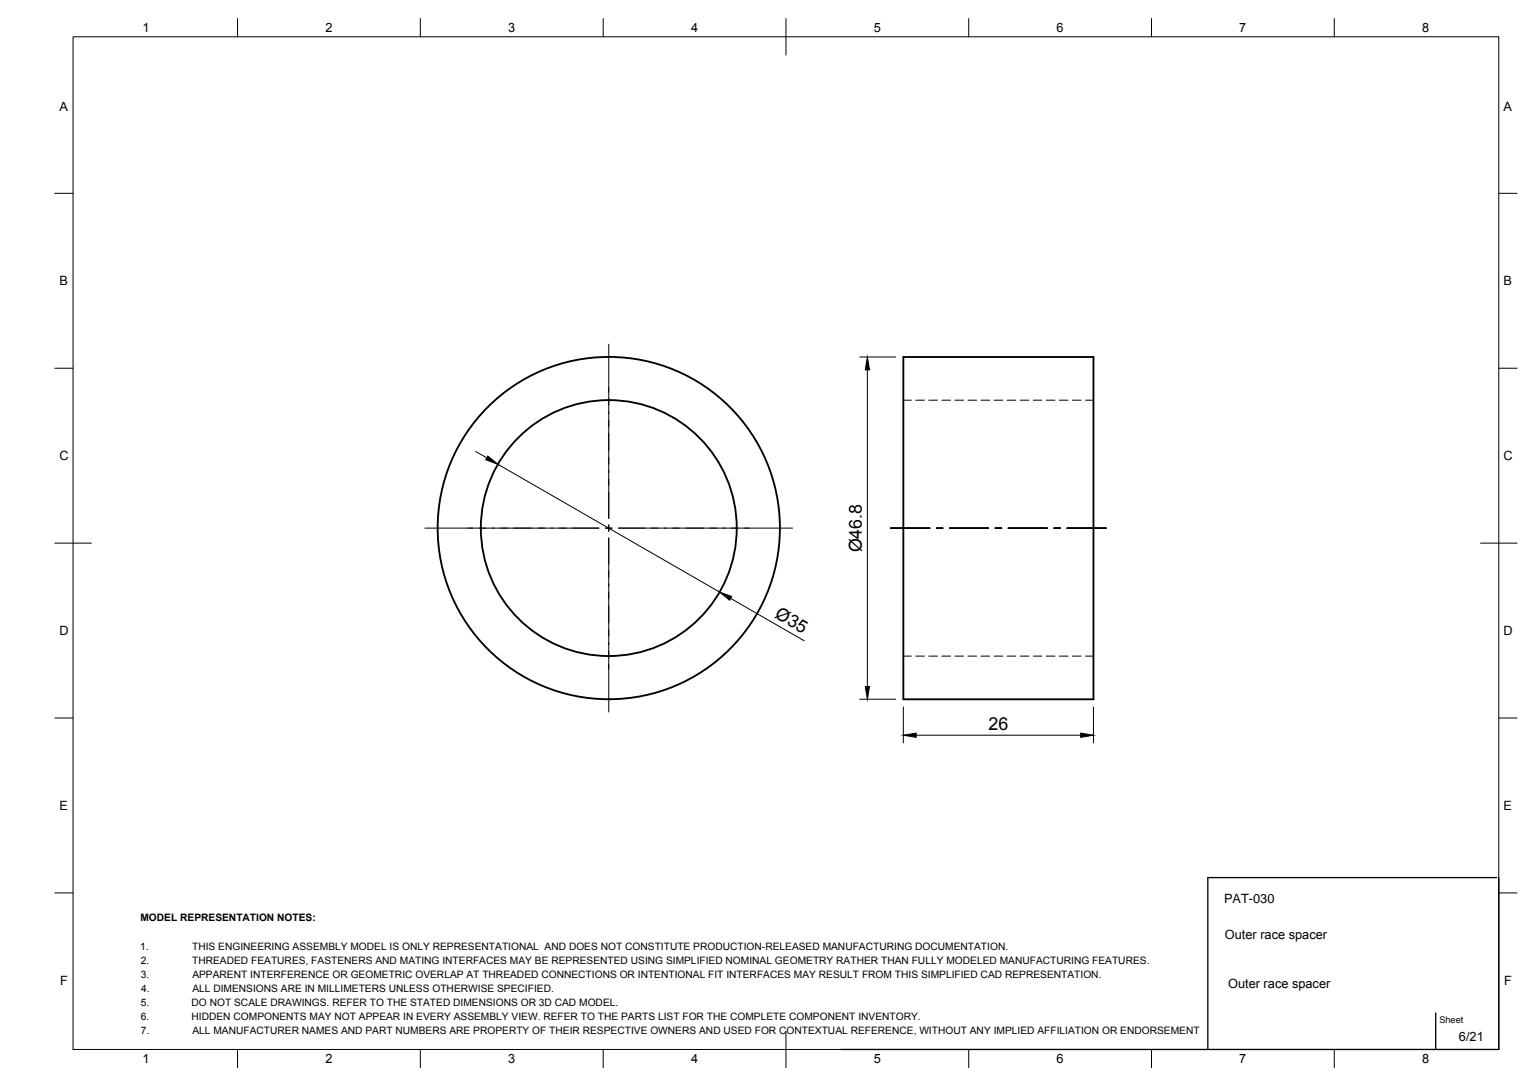
ISO-10303-21;
HEADER;
/* Generated by software containing ST-Developer
 * from STEP Tools, Inc. (www.steptools.com) 
 */

FILE_DESCRIPTION(
/* description */ ('Double-bearing flanged cartridge'),
/* implementation_level */ '2;1');

FILE_NAME(
/* name */ 'Outer race spacer.step',
/* time_stamp */ '2026-10-28T03:26:40-07:00',
/* author */ (''),
/* organization */ (''),
/* preprocessor_version */ 'ST-DEVELOPER v20.2',
/* originating_system */ 'Autodesk Translation Framework v15.17.0.0',
/* authorisation */ '');

FILE_SCHEMA (('AUTOMOTIVE_DESIGN { 1 0 10303 214 3 1 1 }'));
ENDSEC;

DATA;
#10=MECHANICAL_DESIGN_GEOMETRIC_PRESENTATION_REPRESENTATION('',(#204),#5535);
#168=SHAPE_REPRESENTATION_RELATIONSHIP('SRR','None',#5610,#182);
#182=ADVANCED_BREP_SHAPE_REPRESENTATION('',(#226),#5526);
#204=STYLED_ITEM('',(#5764),#226);
#226=MANIFOLD_SOLID_BREP('Body1',#2338);
#262=FACE_BOUND('',#621,.T.);
#263=FACE_BOUND('',#623,.T.);
#329=PLANE('',#2706);
#330=PLANE('',#2707);
#440=FACE_OUTER_BOUND('',#618,.T.);
#441=FACE_OUTER_BOUND('',#619,.T.);
#442=FACE_OUTER_BOUND('',#620,.T.);
#443=FACE_OUTER_BOUND('',#622,.T.);
#618=EDGE_LOOP('',(#1858,#1859,#1860,#1861));
#619=EDGE_LOOP('',(#1862,#1863,#1864,#1865));
#620=EDGE_LOOP('',(#1866));
#621=EDGE_LOOP('',(#1867));
#622=EDGE_LOOP('',(#1868));
#623=EDGE_LOOP('',(#1869));
#758=LINE('',#4385,#844);
#759=LINE('',#4391,#845);
#844=VECTOR('',#3299,1.75);
#845=VECTOR('',#3306,2.34);
#1002=CIRCLE('',#2701,1.75);
#1003=CIRCLE('',#2702,1.75);
#1004=CIRCLE('',#2704,2.34);
#1005=CIRCLE('',#2705,2.34);
#1184=VERTEX_POINT('',#4382);
#1185=VERTEX_POINT('',#4384);
#1186=VERTEX_POINT('',#4388);
#1187=VERTEX_POINT('',#4390);
#1422=EDGE_CURVE('',#1184,#1184,#1002,.T.);
#1423=EDGE_CURVE('',#1184,#1185,#758,.T.);
#1424=EDGE_CURVE('',#1185,#1185,#1003,.T.);
#1425=EDGE_CURVE('',#1186,#1186,#1004,.T.);
#1426=EDGE_CURVE('',#1186,#1187,#759,.T.);
#1427=EDGE_CURVE('',#1187,#1187,#1005,.T.);
#1858=ORIENTED_EDGE('',*,*,#1422,.F.);
#1859=ORIENTED_EDGE('',*,*,#1423,.T.);
#1860=ORIENTED_EDGE('',*,*,#1424,.T.);
#1861=ORIENTED_EDGE('',*,*,#1423,.F.);
#1862=ORIENTED_EDGE('',*,*,#1425,.F.);
#1863=ORIENTED_EDGE('',*,*,#1426,.T.);
#1864=ORIENTED_EDGE('',*,*,#1427,.T.);
#1865=ORIENTED_EDGE('',*,*,#1426,.F.);
#1866=ORIENTED_EDGE('',*,*,#1425,.T.);
#1867=ORIENTED_EDGE('',*,*,#1422,.T.);
#1868=ORIENTED_EDGE('',*,*,#1427,.F.);
#1869=ORIENTED_EDGE('',*,*,#1424,.F.);
#2142=CYLINDRICAL_SURFACE('',#2700,1.75);
#2143=CYLINDRICAL_SURFACE('',#2703,2.34);
#2254=ADVANCED_FACE('',(#440),#2142,.F.);
#2255=ADVANCED_FACE('',(#441),#2143,.T.);
#2256=ADVANCED_FACE('',(#442,#262),#329,.T.);
#2257=ADVANCED_FACE('',(#443,#263),#330,.F.);
#2338=CLOSED_SHELL('',(#2254,#2255,#2256,#2257));
#2699=AXIS2_PLACEMENT_3D('',#4380,#3293,#3294);
#2700=AXIS2_PLACEMENT_3D('',#4381,#3295,#3296);
#2701=AXIS2_PLACEMENT_3D('',#4383,#3297,#3298);
#2702=AXIS2_PLACEMENT_3D('',#4386,#3300,#3301);
#2703=AXIS2_PLACEMENT_3D('',#4387,#3302,#3303);
#2704=AXIS2_PLACEMENT_3D('',#4389,#3304,#3305);
#2705=AXIS2_PLACEMENT_3D('',#4392,#3307,#3308);
#2706=AXIS2_PLACEMENT_3D('',#4393,#3309,#3310);
#2707=AXIS2_PLACEMENT_3D('',#4394,#3311,#3312);
#3293=DIRECTION('axis',(0.,0.,1.));
#3294=DIRECTION('refdir',(1.,0.,0.));
#3295=DIRECTION('center_axis',(0.,1.,0.));
#3296=DIRECTION('ref_axis',(1.,0.,0.));
#3297=DIRECTION('center_axis',(0.,-1.,0.));
#3298=DIRECTION('ref_axis',(1.,0.,0.));
#3299=DIRECTION('',(0.,-1.,0.));
#3300=DIRECTION('center_axis',(0.,-1.,0.));
#3301=DIRECTION('ref_axis',(1.,0.,0.));
#3302=DIRECTION('center_axis',(0.,1.,0.));
#3303=DIRECTION('ref_axis',(1.,0.,0.));
#3304=DIRECTION('center_axis',(0.,1.,0.));
#3305=DIRECTION('ref_axis',(1.,0.,0.));
#3306=DIRECTION('',(0.,-1.,0.));
#3307=DIRECTION('center_axis',(0.,1.,0.));
#3308=DIRECTION('ref_axis',(1.,0.,0.));
#3309=DIRECTION('center_axis',(0.,1.,0.));
#3310=DIRECTION('ref_axis',(1.,0.,0.));
#3311=DIRECTION('center_axis',(0.,1.,0.));
#3312=DIRECTION('ref_axis',(1.,0.,0.));
#4380=CARTESIAN_POINT('',(0.,0.,0.));
#4381=CARTESIAN_POINT('Origin',(0.,1.7,4.5));
#4382=CARTESIAN_POINT('',(-1.75,4.3,4.5));
#4383=CARTESIAN_POINT('Origin',(0.,4.3,4.5));
#4384=CARTESIAN_POINT('',(-1.75,1.7,4.5));
#4385=CARTESIAN_POINT('',(-1.75,1.7,4.5));
#4386=CARTESIAN_POINT('Origin',(0.,1.7,4.5));
#4387=CARTESIAN_POINT('Origin',(0.,1.7,4.5));
#4388=CARTESIAN_POINT('',(-2.34,4.3,4.5));
#4389=CARTESIAN_POINT('Origin',(0.,4.3,4.5));
#4390=CARTESIAN_POINT('',(-2.34,1.7,4.5));
#4391=CARTESIAN_POINT('',(-2.34,1.7,4.5));
#4392=CARTESIAN_POINT('Origin',(0.,1.7,4.5));
#4393=CARTESIAN_POINT('Origin',(0.,4.3,4.5));
#4394=CARTESIAN_POINT('Origin',(0.,1.7,4.5));
#5507=UNCERTAINTY_MEASURE_WITH_UNIT(LENGTH_MEASURE(0.001),#5536,
'DISTANCE_ACCURACY_VALUE',
'Maximum model space distance between geometric entities at asserted c
onnectivities');
#5516=UNCERTAINTY_MEASURE_WITH_UNIT(LENGTH_MEASURE(0.001),#5536,
'DISTANCE_ACCURACY_VALUE',
'Maximum model space distance between geometric entities at asserted c
onnectivities');
#5526=(
GEOMETRIC_REPRESENTATION_CONTEXT(3)
GLOBAL_UNCERTAINTY_ASSIGNED_CONTEXT((#5507))
GLOBAL_UNIT_ASSIGNED_CONTEXT((#5536,#5538,#5539))
REPRESENTATION_CONTEXT('','3D')
);
#5535=(
GEOMETRIC_REPRESENTATION_CONTEXT(3)
GLOBAL_UNCERTAINTY_ASSIGNED_CONTEXT((#5516))
GLOBAL_UNIT_ASSIGNED_CONTEXT((#5536,#5538,#5539))
REPRESENTATION_CONTEXT('','3D')
);
#5536=(
LENGTH_UNIT()
NAMED_UNIT(*)
SI_UNIT(.CENTI.,.METRE.)
);
#5538=(
NAMED_UNIT(*)
PLANE_ANGLE_UNIT()
SI_UNIT($,.RADIAN.)
);
#5539=(
NAMED_UNIT(*)
SI_UNIT($,.STERADIAN.)
SOLID_ANGLE_UNIT()
);
#5549=SHAPE_DEFINITION_REPRESENTATION(#5572,#5610);
#5572=PRODUCT_DEFINITION_SHAPE('',$,#5629);
#5610=SHAPE_REPRESENTATION('',(#2699),#5526);
#5619=PRODUCT_DEFINITION_CONTEXT('part definition',#5675,'design');
#5629=PRODUCT_DEFINITION('Outer race spacer','Outer race spacer',#5647,
#5619);
#5647=PRODUCT_DEFINITION_FORMATION('',$,#5686);
#5675=APPLICATION_CONTEXT(
'Core Data for Automotive Mechanical Design Process');
#5676=PRODUCT_CONTEXT('part definition',#5675,'mechanical');
#5686=PRODUCT('Outer race spacer','Outer race spacer',
'Outer race spacer',(#5676));
#5758=COLOUR_RGB('Grey',0.48,0.52,0.57);
#5759=FILL_AREA_STYLE_COLOUR('',#5758);
#5760=FILL_AREA_STYLE('',(#5759));
#5761=SURFACE_STYLE_FILL_AREA(#5760);
#5762=SURFACE_SIDE_STYLE('',(#5761));
#5763=SURFACE_STYLE_USAGE(.BOTH.,#5762);
#5764=PRESENTATION_STYLE_ASSIGNMENT((#5763));
ENDSEC;
END-ISO-10303-21;
